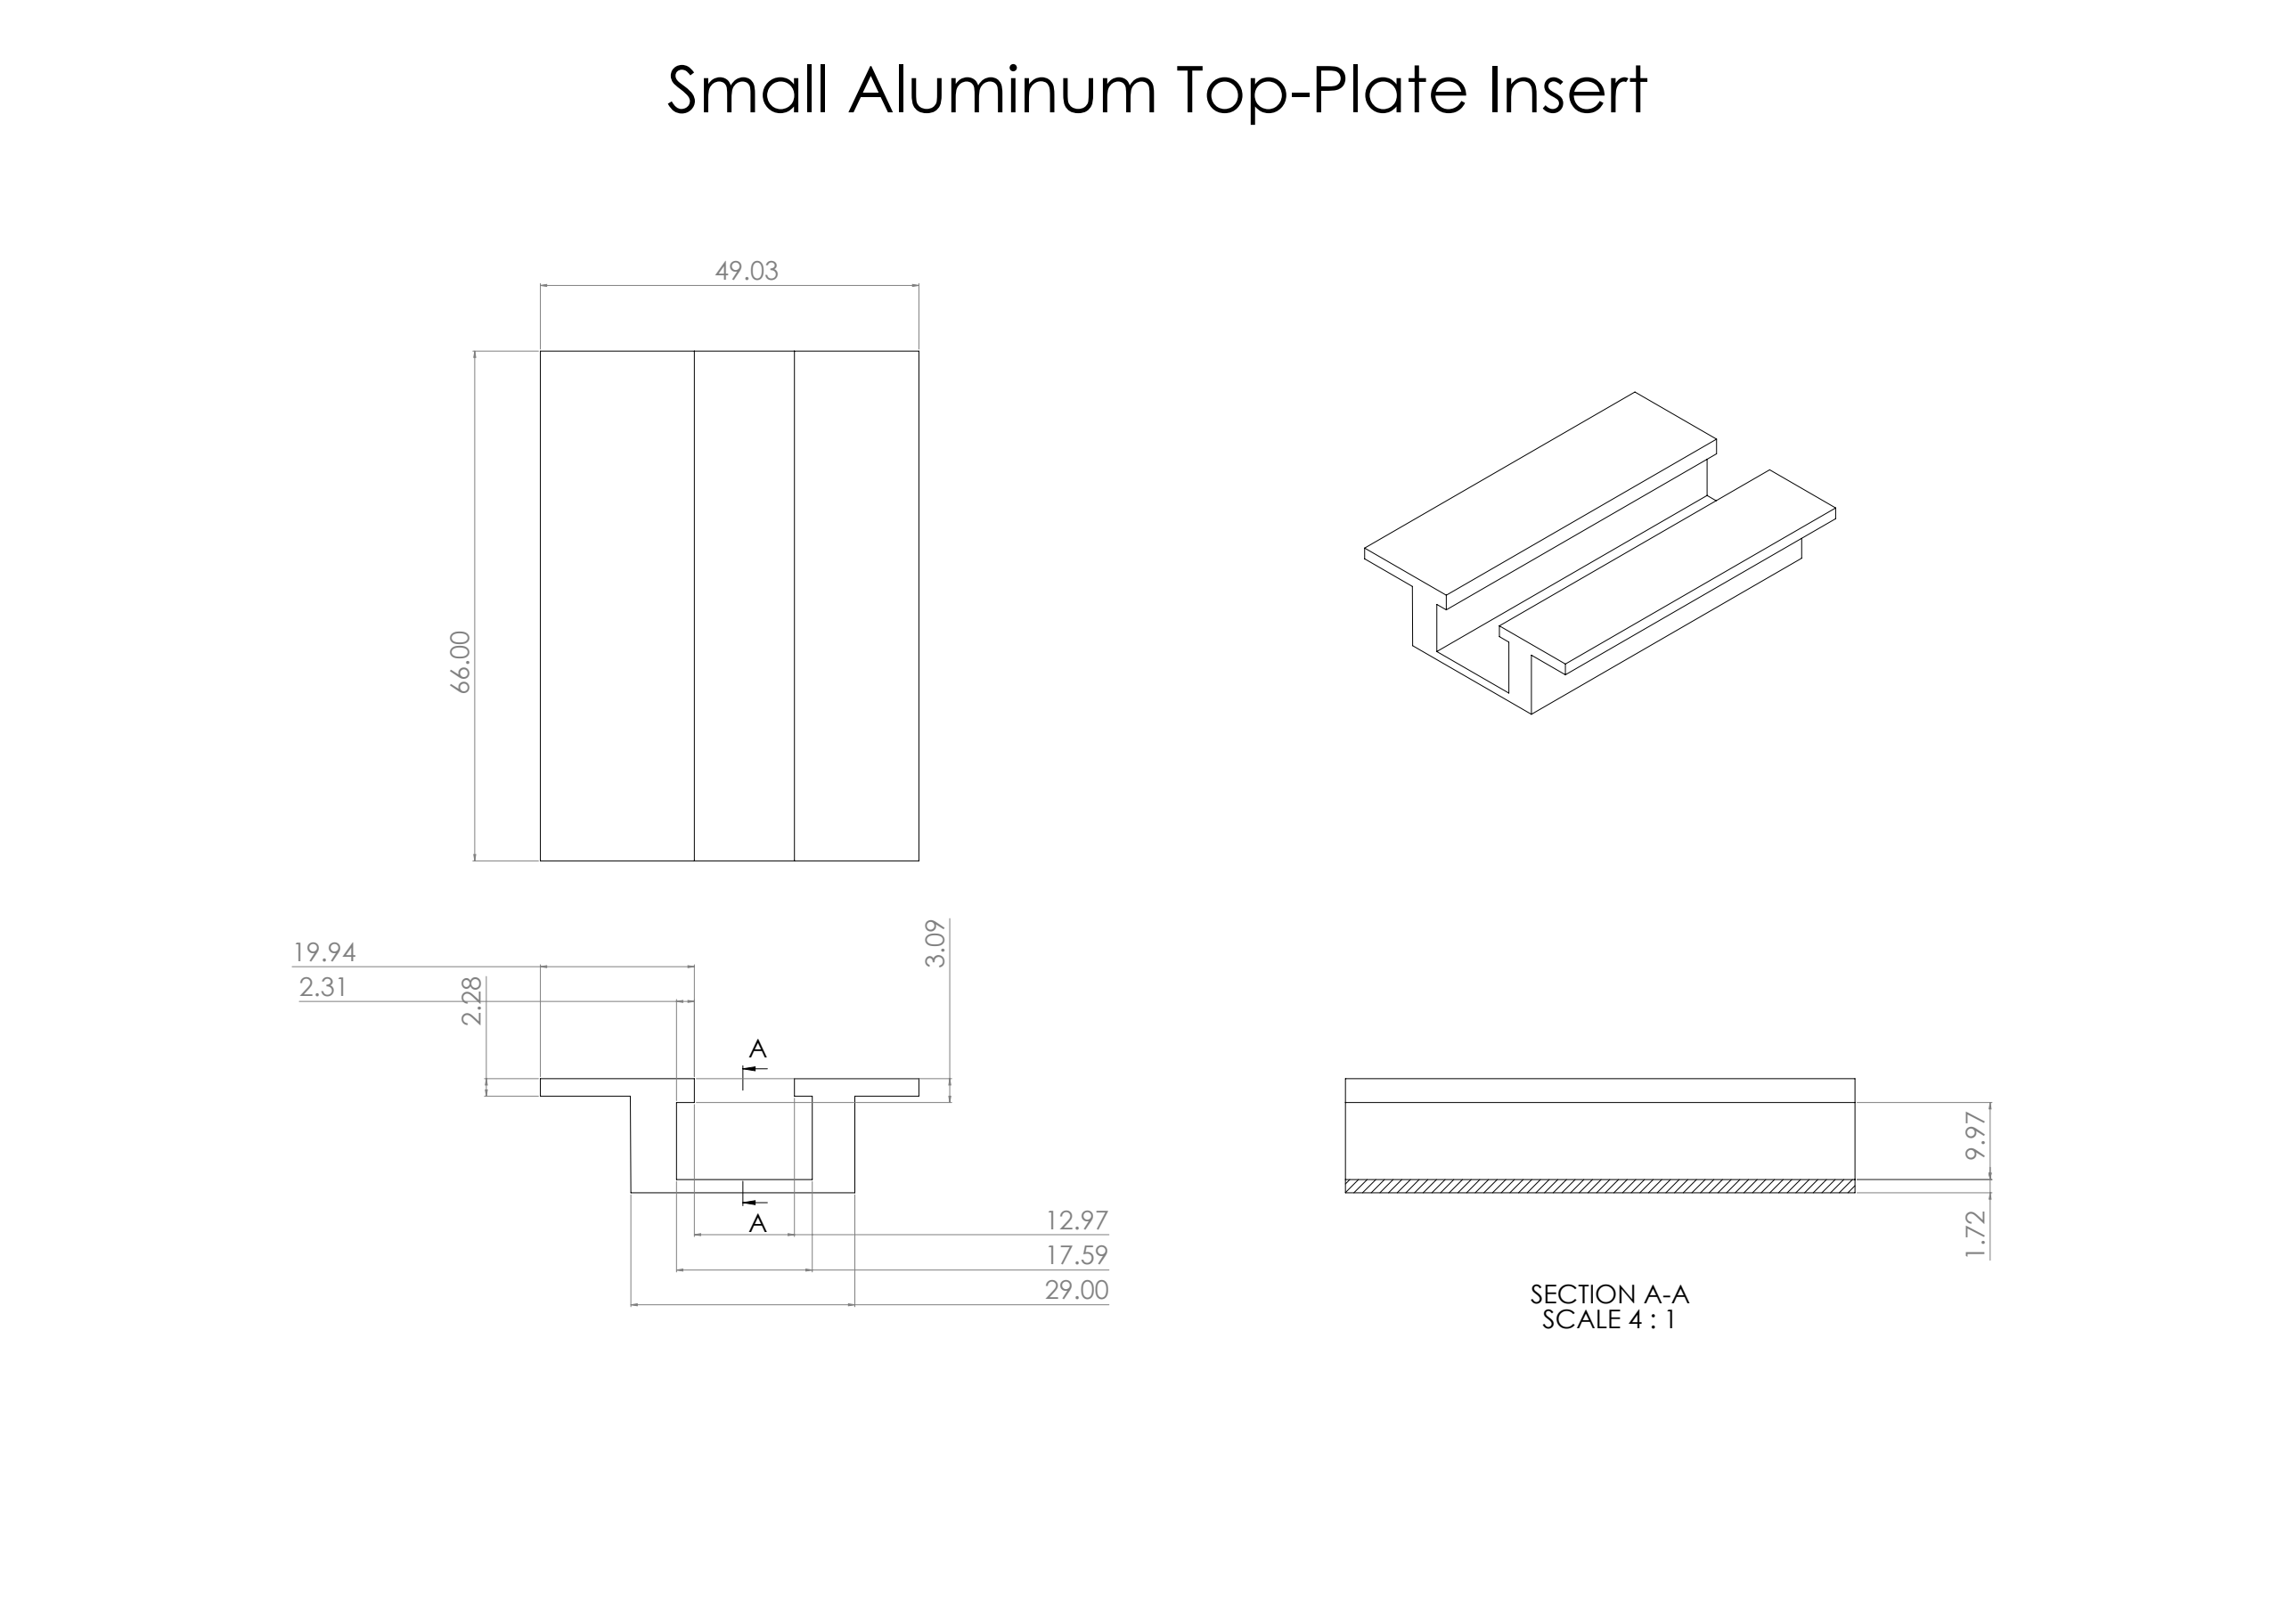
ISO-10303-21;
HEADER;
FILE_DESCRIPTION (('STEP AP214'),
    '1' );
FILE_NAME ('Small Aluminum Top-Plate Insert.step',
    '2026-10-24T21:31:31',
    ( '' ),
    ( '' ),
    'SwSTEP 2.0',
    'SolidWorks 2025',
    '' );
FILE_SCHEMA (( 'AUTOMOTIVE_DESIGN' ));
ENDSEC;

DATA;
#11=EDGE_LOOP ( 'NONE', ( #10298, #886, #9841, #4831, #11174, #11784, #1803, #163, #11627, #11601, #5374, #7472, #708, #12281, #12120, #14505 ) ) ;
#69=LINE ( 'NONE', #10606, #11985 ) ;
#101=ORIENTED_EDGE ( 'NONE', *, *, #8706, .F. ) ;
#123=ADVANCED_FACE ( 'NONE', ( #3273 ), #5820, .F. ) ;
#148=LINE ( 'NONE', #14233, #12794 ) ;
#163=ORIENTED_EDGE ( 'NONE', *, *, #14073, .T. ) ;
#171=VECTOR ( 'NONE', #13826, 1000.000000000000000 ) ;
#187=CARTESIAN_POINT ( 'NONE',  ( 67.21328690825531282, 25.52935533987996664, 84.20452624982236500 ) ) ;
#212=PLANE ( 'NONE',  #10140 ) ;
#275=AXIS2_PLACEMENT_3D ( 'NONE', #4169, #10894, #7496 ) ;
#346=LINE ( 'NONE', #12902, #10507 ) ;
#348=CARTESIAN_POINT ( 'NONE',  ( 96.29968967959054282, 25.52935533987996664, 33.00000000000012790 ) ) ;
#409=EDGE_CURVE ( 'NONE', #4378, #2618, #11532, .T. ) ;
#440=CARTESIAN_POINT ( 'NONE',  ( 96.29968967959054282, 23.25070940071369208, 33.00000000000012790 ) ) ;
#479=EDGE_LOOP ( 'NONE', ( #6850, #11834, #11522, #3223 ) ) ;
#480=CARTESIAN_POINT ( 'NONE',  ( 88.00000000000001421, 10.75070940071369208, -33.00000000000012790 ) ) ;
#488=CARTESIAN_POINT ( 'NONE',  ( 47.27423575335444639, 23.25070940071368852, 84.20452624982236500 ) ) ;
#497=FACE_OUTER_BOUND ( 'NONE', #6933, .T. ) ;
#563=LINE ( 'NONE', #7876, #12055 ) ;
#591=DIRECTION ( 'NONE',  ( -1.000000000000000000, 0.000000000000000000, 0.000000000000000000 ) ) ;
#619=VERTEX_POINT ( 'NONE', #7390 ) ;
#630=AXIS2_PLACEMENT_3D ( 'NONE', #11136, #591, #8901 ) ;
#654=ADVANCED_FACE ( 'NONE', ( #5008 ), #9713, .F. ) ;
#676=VECTOR ( 'NONE', #14030, 1000.000000000000000 ) ;
#698=DIRECTION ( 'NONE',  ( 0.000000000000000000, -1.000000000000000000, 0.000000000000000000 ) ) ;
#708=ORIENTED_EDGE ( 'NONE', *, *, #10704, .T. ) ;
#734=CARTESIAN_POINT ( 'NONE',  ( 67.21328690825531282, 25.52935533987996664, -33.00000000000012790 ) ) ;
#750=VERTEX_POINT ( 'NONE', #6949 ) ;
#765=DIRECTION ( 'NONE',  ( 0.000000000000000000, -1.000000000000000000, 0.000000000000000000 ) ) ;
#770=VECTOR ( 'NONE', #9472, 1000.000000000000000 ) ;
#788=VERTEX_POINT ( 'NONE', #4558 ) ;
#803=VECTOR ( 'NONE', #6520, 1000.000000000000000 ) ;
#823=CARTESIAN_POINT ( 'NONE',  ( 80.18290120114222930, 25.52935533987996664, 84.20452624982236500 ) ) ;
#848=ORIENTED_EDGE ( 'NONE', *, *, #10704, .F. ) ;
#878=CARTESIAN_POINT ( 'NONE',  ( 82.49066175147797253, 12.46743062497963450, -33.00000000000012790 ) ) ;
#886=ORIENTED_EDGE ( 'NONE', *, *, #4268, .T. ) ;
#895=VECTOR ( 'NONE', #2862, 1000.000000000000000 ) ;
#923=VECTOR ( 'NONE', #12640, 1000.000000000000000 ) ;
#929=SHAPE_REPRESENTATION_RELATIONSHIP ( 'NONE' , 'NONE' ,  #2449, #8343 ) ;
#949=EDGE_CURVE ( 'NONE', #3754, #3249, #2996, .T. ) ;
#962=AXIS2_PLACEMENT_3D ( 'NONE', #12322, #765, #7710 ) ;
#969=EDGE_CURVE ( 'NONE', #12642, #2618, #1832, .T. ) ;
#1004=STYLED_ITEM('',(#15279),#4097);
#1041=VECTOR ( 'NONE', #698, 1000.000000000000000 ) ;
#1096=VERTEX_POINT ( 'NONE', #9302 ) ;
#1101=LINE ( 'NONE', #5813, #11583 ) ;
#1148=CARTESIAN_POINT ( 'NONE',  ( 88.00000000000000000, 23.25070940071369208, -33.00000000000012790 ) ) ;
#1158=DIRECTION ( 'NONE',  ( -1.110223024625156540E-15, 1.000000000000000000, 0.000000000000000000 ) ) ;
#1177=EDGE_CURVE ( 'NONE', #9470, #12642, #1669, .T. ) ;
#1199=PRODUCT_DEFINITION ( 'UNKNOWN', '', #11005, #4748 ) ;
#1215=ORIENTED_EDGE ( 'NONE', *, *, #949, .F. ) ;
#1218=ORIENTED_EDGE ( 'NONE', *, *, #5311, .F. ) ;
#1279=PLANE ( 'NONE',  #11718 ) ;
#1339=LINE ( 'NONE', #187, #12832 ) ;
#1347=DIRECTION ( 'NONE',  ( -0.000000000000000000, -0.000000000000000000, -1.000000000000000000 ) ) ;
#1354=ORIENTED_EDGE ( 'NONE', *, *, #14964, .T. ) ;
#1356=ORIENTED_EDGE ( 'NONE', *, *, #9741, .T. ) ;
#1369=CARTESIAN_POINT ( 'NONE',  ( 59.06137132172460014, 0.3483485318593032565, -33.00000000000012790 ) ) ;
#1378=ORIENTED_EDGE ( 'NONE', *, *, #14002, .T. ) ;
#1387=ADVANCED_FACE ( 'NONE', ( #12279 ), #6653, .F. ) ;
#1433=EDGE_LOOP ( 'NONE', ( #6266, #13083, #3751, #10819 ) ) ;
#1441=VERTEX_POINT ( 'NONE', #10128 ) ;
#1474=VERTEX_POINT ( 'NONE', #878 ) ;
#1497=LINE ( 'NONE', #348, #6923 ) ;
#1509=ORIENTED_EDGE ( 'NONE', *, *, #11188, .T. ) ;
#1516=ORIENTED_EDGE ( 'NONE', *, *, #409, .F. ) ;
#1536=LINE ( 'NONE', #2764, #13361 ) ;
#1538=VECTOR ( 'NONE', #4607, 1000.000000000000000 ) ;
#1539=VECTOR ( 'NONE', #8765, 1000.000000000000000 ) ;
#1541=ORIENTED_EDGE ( 'NONE', *, *, #13654, .F. ) ;
#1562=CARTESIAN_POINT ( 'NONE',  ( 67.21328690825531282, 22.43695620243006772, -33.00000000000012790 ) ) ;
#1586=CARTESIAN_POINT ( 'NONE',  ( 58.92629142760363692, 23.25070940071368852, 84.20452624982236500 ) ) ;
#1598=ORIENTED_EDGE ( 'NONE', *, *, #5035, .T. ) ;
#1660=PLANE ( 'NONE',  #10735 ) ;
#1669=LINE ( 'NONE', #12057, #6239 ) ;
#1709=DIRECTION ( 'NONE',  ( -1.000000000000000000, -1.156482317317871725E-16, 0.000000000000000000 ) ) ;
#1739=EDGE_CURVE ( 'NONE', #6140, #7395, #10489, .T. ) ;
#1803=ORIENTED_EDGE ( 'NONE', *, *, #5053, .T. ) ;
#1832=LINE ( 'NONE', #823, #803 ) ;
#1899=ORIENTED_EDGE ( 'NONE', *, *, #14964, .F. ) ;
#1930=ORIENTED_EDGE ( 'NONE', *, *, #9241, .F. ) ;
#1931=( NAMED_UNIT ( * ) PLANE_ANGLE_UNIT ( ) SI_UNIT ( $, .RADIAN. ) );
#1947=DIRECTION ( 'NONE',  ( -0.000000000000000000, -0.000000000000000000, -1.000000000000000000 ) ) ;
#1949=VECTOR ( 'NONE', #5608, 1000.000000000000000 ) ;
#1954=DIRECTION ( 'NONE',  ( 0.000000000000000000, -1.000000000000000000, 0.000000000000000000 ) ) ;
#1969=EDGE_CURVE ( 'NONE', #11430, #3386, #11495, .T. ) ;
#1982=ORIENTED_EDGE ( 'NONE', *, *, #1177, .F. ) ;
#1986=VECTOR ( 'NONE', #11667, 1000.000000000000000 ) ;
#2001=APPLICATION_CONTEXT ( 'automotive_design' ) ;
#2023=EDGE_LOOP ( 'NONE', ( #2080, #1378, #2516, #4174 ) ) ;
#2048=ORIENTED_EDGE ( 'NONE', *, *, #14002, .F. ) ;
#2065=ORIENTED_EDGE ( 'NONE', *, *, #2181, .T. ) ;
#2071=CARTESIAN_POINT ( 'NONE',  ( 96.29968967959054282, 25.52935533987996664, -33.00000000000012790 ) ) ;
#2080=ORIENTED_EDGE ( 'NONE', *, *, #9815, .F. ) ;
#2129=( GEOMETRIC_REPRESENTATION_CONTEXT ( 3 ) GLOBAL_UNCERTAINTY_ASSIGNED_CONTEXT ( ( #13980 ) ) GLOBAL_UNIT_ASSIGNED_CONTEXT ( ( #12561, #1931, #12718 ) ) REPRESENTATION_CONTEXT ( 'NONE', 'WORKASPACE' ) );
#2181=EDGE_CURVE ( 'NONE', #9470, #5069, #5821, .T. ) ;
#2237=ORIENTED_EDGE ( 'NONE', *, *, #6729, .T. ) ;
#2276=VECTOR ( 'NONE', #5661, 1000.000000000000000 ) ;
#2347=DIRECTION ( 'NONE',  ( 0.000000000000000000, 0.000000000000000000, 1.000000000000000000 ) ) ;
#2363=CARTESIAN_POINT ( 'NONE',  ( 57.92627403409715470, 23.25070940071368852, -33.00000000000012790 ) ) ;
#2366=ORIENTED_EDGE ( 'NONE', *, *, #14128, .F. ) ;
#2443=APPLICATION_CONTEXT ( 'automotive_design' ) ;
#2449=SHAPE_REPRESENTATION ( 'Small Aluminum Top-Plate Insert', ( #6315 ), #2129 ) ;
#2461=CARTESIAN_POINT ( 'NONE',  ( 64.90552635791956959, 12.46743062497963450, -33.00000000000012790 ) ) ;
#2516=ORIENTED_EDGE ( 'NONE', *, *, #9344, .F. ) ;
#2553=AXIS2_PLACEMENT_3D ( 'NONE', #10050, #14815, #4114 ) ;
#2618=VERTEX_POINT ( 'NONE', #6600 ) ;
#2656=EDGE_CURVE ( 'NONE', #9890, #6001, #8753, .T. ) ;
#2722=DIRECTION ( 'NONE',  ( 0.000000000000000000, -1.000000000000000000, 0.000000000000000000 ) ) ;
#2764=CARTESIAN_POINT ( 'NONE',  ( 67.21328690825531282, 25.52935533987996664, 33.00000000000012790 ) ) ;
#2799=LINE ( 'NONE', #7492, #3177 ) ;
#2814=CARTESIAN_POINT ( 'NONE',  ( 82.49066175147797253, 23.25070940071369208, -33.00000000000012790 ) ) ;
#2862=DIRECTION ( 'NONE',  ( -0.000000000000000000, -0.000000000000000000, -1.000000000000000000 ) ) ;
#2867=PLANE ( 'NONE',  #10844 ) ;
#2887=VERTEX_POINT ( 'NONE', #8441 ) ;
#2913=DIRECTION ( 'NONE',  ( -1.000000000000000000, 0.000000000000000000, 0.000000000000000000 ) ) ;
#2942=ADVANCED_FACE ( 'NONE', ( #8574 ), #14429, .F. ) ;
#2951=ADVANCED_FACE ( 'NONE', ( #13565 ), #2867, .F. ) ;
#2964=ORIENTED_EDGE ( 'NONE', *, *, #7226, .F. ) ;
#2966=DIRECTION ( 'NONE',  ( -0.000000000000000000, 0.000000000000000000, 1.000000000000000000 ) ) ;
#2981=ORIENTED_EDGE ( 'NONE', *, *, #4998, .F. ) ;
#2996=LINE ( 'NONE', #5610, #10659 ) ;
#3008=ADVANCED_FACE ( 'NONE', ( #4019 ), #7425, .F. ) ;
#3038=DIRECTION ( 'NONE',  ( 0.000000000000000000, 0.000000000000000000, 1.000000000000000000 ) ) ;
#3087=CARTESIAN_POINT ( 'NONE',  ( 88.00000000000001421, 10.75070940071369208, 33.00000000000012790 ) ) ;
#3092=CARTESIAN_POINT ( 'NONE',  ( 47.27423575335444639, 23.25070940071368852, 33.00000000000012790 ) ) ;
#3172=VERTEX_POINT ( 'NONE', #10649 ) ;
#3177=VECTOR ( 'NONE', #12177, 1000.000000000000000 ) ;
#3223=ORIENTED_EDGE ( 'NONE', *, *, #6729, .F. ) ;
#3249=VERTEX_POINT ( 'NONE', #8268 ) ;
#3270=DIRECTION ( 'NONE',  ( -1.000000000000000000, 0.000000000000000000, 0.000000000000000000 ) ) ;
#3273=FACE_OUTER_BOUND ( 'NONE', #9368, .T. ) ;
#3290=DIRECTION ( 'NONE',  ( -0.005897974685767391929, 0.9999826067960413400, 0.000000000000000000 ) ) ;
#3293=LINE ( 'NONE', #13605, #1949 ) ;
#3386=VERTEX_POINT ( 'NONE', #1562 ) ;
#3462=PLANE ( 'NONE',  #6224 ) ;
#3465=LINE ( 'NONE', #1148, #770 ) ;
#3528=ADVANCED_FACE ( 'NONE', ( #12252 ), #6539, .F. ) ;
#3591=DIRECTION ( 'NONE',  ( 0.000000000000000000, 1.000000000000000000, -0.000000000000000000 ) ) ;
#3624=ORIENTED_EDGE ( 'NONE', *, *, #2656, .T. ) ;
#3677=EDGE_CURVE ( 'NONE', #3754, #788, #9224, .T. ) ;
#3690=EDGE_CURVE ( 'NONE', #6772, #1096, #3293, .T. ) ;
#3723=LINE ( 'NONE', #9670, #895 ) ;
#3751=ORIENTED_EDGE ( 'NONE', *, *, #5035, .F. ) ;
#3754=VERTEX_POINT ( 'NONE', #4438 ) ;
#3811=DIRECTION ( 'NONE',  ( 1.000000000000000000, 0.000000000000000000, 0.000000000000000000 ) ) ;
#3843=ORIENTED_EDGE ( 'NONE', *, *, #8706, .T. ) ;
#3898=CARTESIAN_POINT ( 'NONE',  ( 59.00001739350650354, 10.75070940071368852, 33.00000000000012790 ) ) ;
#3907=DIRECTION ( 'NONE',  ( -0.000000000000000000, -0.000000000000000000, -1.000000000000000000 ) ) ;
#3928=LINE ( 'NONE', #12242, #1539 ) ;
#3991=AXIS2_PLACEMENT_3D ( 'NONE', #6880, #3270, #4258 ) ;
#4019=FACE_OUTER_BOUND ( 'NONE', #7636, .T. ) ;
#4021=EDGE_CURVE ( 'NONE', #6859, #5990, #7026, .T. ) ;
#4024=ORIENTED_EDGE ( 'NONE', *, *, #11631, .T. ) ;
#4039=CARTESIAN_POINT ( 'NONE',  ( 96.29968967959054282, 25.52935533987996664, 84.20452624982236500 ) ) ;
#4059=DIRECTION ( 'NONE',  ( 0.000000000000000000, 1.000000000000000000, -0.000000000000000000 ) ) ;
#4079=EDGE_LOOP ( 'NONE', ( #9449, #4802, #6054, #101 ) ) ;
#4082=CARTESIAN_POINT ( 'NONE',  ( 0.000000000000000000, 0.000000000000000000, 0.000000000000000000 ) ) ;
#4097=MANIFOLD_SOLID_BREP ( 'Move Face2', #11190 ) ;
#4114=DIRECTION ( 'NONE',  ( 0.000000000000000000, -0.000000000000000000, -1.000000000000000000 ) ) ;
#4169=CARTESIAN_POINT ( 'NONE',  ( 88.00000000000000000, 23.25070940071369208, 84.20452624982236500 ) ) ;
#4174=ORIENTED_EDGE ( 'NONE', *, *, #10349, .F. ) ;
#4222=CARTESIAN_POINT ( 'NONE',  ( 82.49066175147797253, 23.25070940071369208, 33.00000000000012790 ) ) ;
#4244=PRODUCT_DEFINITION_SHAPE ( 'NONE', 'NONE',  #1199 ) ;
#4258=DIRECTION ( 'NONE',  ( 0.000000000000000000, 0.000000000000000000, 1.000000000000000000 ) ) ;
#4268=EDGE_CURVE ( 'NONE', #5864, #9470, #1497, .T. ) ;
#4360=VECTOR ( 'NONE', #1954, 1000.000000000000000 ) ;
#4378=VERTEX_POINT ( 'NONE', #11617 ) ;
#4438=CARTESIAN_POINT ( 'NONE',  ( 82.49066175147797253, 23.25070940071369208, 33.00000000000014211 ) ) ;
#4452=DIRECTION ( 'NONE',  ( 1.000000000000000000, -0.000000000000000000, 0.000000000000000000 ) ) ;
#4519=EDGE_CURVE ( 'NONE', #6001, #619, #3465, .T. ) ;
#4558=CARTESIAN_POINT ( 'NONE',  ( 82.49066175147797253, 23.25070940071369208, -33.00000000000012790 ) ) ;
#4564=CARTESIAN_POINT ( 'NONE',  ( 59.00001739350650354, 10.75070940071368852, 84.20452624982236500 ) ) ;
#4588=ORIENTED_EDGE ( 'NONE', *, *, #14888, .F. ) ;
#4607=DIRECTION ( 'NONE',  ( -0.000000000000000000, -0.000000000000000000, -1.000000000000000000 ) ) ;
#4614=DIRECTION ( 'NONE',  ( 1.000000000000000000, -0.000000000000000000, 0.000000000000000000 ) ) ;
#4627=VERTEX_POINT ( 'NONE', #9183 ) ;
#4629=EDGE_CURVE ( 'NONE', #14228, #1441, #10415, .T. ) ;
#4743=VECTOR ( 'NONE', #14648, 1000.000000000000000 ) ;
#4748=PRODUCT_DEFINITION_CONTEXT ( 'detailed design', #2001, 'design' ) ;
#4771=ORIENTED_EDGE ( 'NONE', *, *, #7741, .F. ) ;
#4802=ORIENTED_EDGE ( 'NONE', *, *, #12107, .T. ) ;
#4818=ORIENTED_EDGE ( 'NONE', *, *, #14852, .F. ) ;
#4831=ORIENTED_EDGE ( 'NONE', *, *, #4998, .T. ) ;
#4842=CARTESIAN_POINT ( 'NONE',  ( -16.99999999999998579, -2.249290599286303927, 33.00000000000012790 ) ) ;
#4998=EDGE_CURVE ( 'NONE', #12642, #2887, #3928, .T. ) ;
#5008=FACE_OUTER_BOUND ( 'NONE', #14284, .T. ) ;
#5034=CARTESIAN_POINT ( 'NONE',  ( 80.18290120114222930, 23.25070940071369208, 84.20452624982236500 ) ) ;
#5035=EDGE_CURVE ( 'NONE', #5069, #9890, #6184, .T. ) ;
#5053=EDGE_CURVE ( 'NONE', #3249, #12316, #8697, .T. ) ;
#5069=VERTEX_POINT ( 'NONE', #2071 ) ;
#5087=EDGE_CURVE ( 'NONE', #2887, #3754, #13770, .T. ) ;
#5088=EDGE_LOOP ( 'NONE', ( #2964, #14634, #9945, #10176 ) ) ;
#5127=CARTESIAN_POINT ( 'NONE',  ( 88.00000000000000000, 23.25070940071369208, 33.00000000000014211 ) ) ;
#5133=DIRECTION ( 'NONE',  ( 1.000000000000000000, -0.000000000000000000, 0.000000000000000000 ) ) ;
#5171=ADVANCED_FACE ( 'NONE', ( #11612 ), #3462, .T. ) ;
#5196=CARTESIAN_POINT ( 'NONE',  ( 0.000000000000000000, 0.000000000000000000, -33.00000000000012790 ) ) ;
#5206=ORIENTED_EDGE ( 'NONE', *, *, #409, .T. ) ;
#5209=PLANE ( 'NONE',  #14912 ) ;
#5218=CARTESIAN_POINT ( 'NONE',  ( 64.90552635791956959, 22.43695620243006772, -33.00000000000012790 ) ) ;
#5231=PLANE ( 'NONE',  #13467 ) ;
#5276=DIRECTION ( 'NONE',  ( 1.000000000000000000, 0.000000000000000000, 0.000000000000000000 ) ) ;
#5311=EDGE_CURVE ( 'NONE', #1096, #14996, #1536, .T. ) ;
#5326=EDGE_CURVE ( 'NONE', #750, #4627, #6374, .T. ) ;
#5352=CARTESIAN_POINT ( 'NONE',  ( 67.21328690825531282, 25.52935533987996664, -33.00000000000012790 ) ) ;
#5374=ORIENTED_EDGE ( 'NONE', *, *, #9815, .T. ) ;
#5447=CARTESIAN_POINT ( 'NONE',  ( 58.99998260679605266, 10.75660737539945622, 84.20452624982236500 ) ) ;
#5466=VECTOR ( 'NONE', #6324, 1000.000000000000000 ) ;
#5510=CARTESIAN_POINT ( 'NONE',  ( 80.18290120114222930, 25.52935533987996664, -33.00000000000012790 ) ) ;
#5562=ORIENTED_EDGE ( 'NONE', *, *, #14852, .T. ) ;
#5605=DIRECTION ( 'NONE',  ( 0.9999826067960413400, 0.005897974685767391929, -0.000000000000000000 ) ) ;
#5608=DIRECTION ( 'NONE',  ( 1.000000000000000000, -0.000000000000000000, 0.000000000000000000 ) ) ;
#5610=CARTESIAN_POINT ( 'NONE',  ( 82.49066175147797253, 12.46743062497963450, 33.00000000000012790 ) ) ;
#5646=DIRECTION ( 'NONE',  ( 0.005897974685767391929, -0.9999826067960413400, 0.000000000000000000 ) ) ;
#5661=DIRECTION ( 'NONE',  ( 1.000000000000000000, -0.000000000000000000, 0.000000000000000000 ) ) ;
#5671=VECTOR ( 'NONE', #14857, 1000.000000000000000 ) ;
#5715=CARTESIAN_POINT ( 'NONE',  ( 88.00000000000000000, 23.25070940071369208, 33.00000000000012790 ) ) ;
#5747=PLANE ( 'NONE',  #3991 ) ;
#5767=CARTESIAN_POINT ( 'NONE',  ( 47.27423575335444639, 25.52935533987996664, 33.00000000000012790 ) ) ;
#5813=CARTESIAN_POINT ( 'NONE',  ( 64.90552635791956959, 22.43695620243006772, 33.00000000000012790 ) ) ;
#5820=PLANE ( 'NONE',  #6330 ) ;
#5821=LINE ( 'NONE', #15203, #13975 ) ;
#5831=VECTOR ( 'NONE', #3907, 1000.000000000000000 ) ;
#5864=VERTEX_POINT ( 'NONE', #13259 ) ;
#5913=ORIENTED_EDGE ( 'NONE', *, *, #3677, .T. ) ;
#5990=VERTEX_POINT ( 'NONE', #6476 ) ;
#6001=VERTEX_POINT ( 'NONE', #6395 ) ;
#6043=PLANE ( 'NONE',  #13108 ) ;
#6054=ORIENTED_EDGE ( 'NONE', *, *, #8949, .F. ) ;
#6137=EDGE_LOOP ( 'NONE', ( #6525, #11863, #13007, #14651 ) ) ;
#6140=VERTEX_POINT ( 'NONE', #11696 ) ;
#6161=LINE ( 'NONE', #6240, #5831 ) ;
#6184=LINE ( 'NONE', #10870, #5466 ) ;
#6186=VECTOR ( 'NONE', #2913, 1000.000000000000000 ) ;
#6219=LINE ( 'NONE', #1586, #4743 ) ;
#6224=AXIS2_PLACEMENT_3D ( 'NONE', #4842, #14160, #8159 ) ;
#6239=VECTOR ( 'NONE', #8665, 1000.000000000000000 ) ;
#6240=CARTESIAN_POINT ( 'NONE',  ( 88.00000000000001421, 10.75070940071369208, 84.20452624982236500 ) ) ;
#6266=ORIENTED_EDGE ( 'NONE', *, *, #4268, .F. ) ;
#6315=AXIS2_PLACEMENT_3D ( 'NONE', #4082, #8567, #11096 ) ;
#6324=DIRECTION ( 'NONE',  ( 0.000000000000000000, -1.000000000000000000, 0.000000000000000000 ) ) ;
#6330=AXIS2_PLACEMENT_3D ( 'NONE', #10282, #9356, #2347 ) ;
#6374=LINE ( 'NONE', #5218, #9407 ) ;
#6383=FACE_OUTER_BOUND ( 'NONE', #4079, .T. ) ;
#6395=CARTESIAN_POINT ( 'NONE',  ( 88.00000000000000000, 23.25070940071369208, -33.00000000000012790 ) ) ;
#6411=DIRECTION ( 'NONE',  ( 1.000000000000000000, 0.000000000000000000, 0.000000000000000000 ) ) ;
#6476=CARTESIAN_POINT ( 'NONE',  ( 59.00001739350650354, 10.75070940071368852, -33.00000000000012790 ) ) ;
#6520=DIRECTION ( 'NONE',  ( -0.000000000000000000, -0.000000000000000000, -1.000000000000000000 ) ) ;
#6525=ORIENTED_EDGE ( 'NONE', *, *, #14073, .F. ) ;
#6539=PLANE ( 'NONE',  #962 ) ;
#6600=CARTESIAN_POINT ( 'NONE',  ( 80.18290120114222930, 25.52935533987996664, -33.00000000000014211 ) ) ;
#6607=CARTESIAN_POINT ( 'NONE',  ( 64.90552635791956959, 12.46743062497963450, 84.20452624982236500 ) ) ;
#6653=PLANE ( 'NONE',  #2553 ) ;
#6729=EDGE_CURVE ( 'NONE', #1441, #6140, #69, .T. ) ;
#6746=ORIENTED_EDGE ( 'NONE', *, *, #4021, .T. ) ;
#6772=VERTEX_POINT ( 'NONE', #14379 ) ;
#6774=LINE ( 'NONE', #5715, #14186 ) ;
#6787=CARTESIAN_POINT ( 'NONE',  ( 58.99998260679605266, 10.75660737539945622, 33.00000000000012790 ) ) ;
#6850=ORIENTED_EDGE ( 'NONE', *, *, #4629, .F. ) ;
#6859=VERTEX_POINT ( 'NONE', #3898 ) ;
#6880=CARTESIAN_POINT ( 'NONE',  ( 67.21328690825531282, 25.52935533987996664, 84.20452624982236500 ) ) ;
#6923=VECTOR ( 'NONE', #10962, 1000.000000000000000 ) ;
#6933=EDGE_LOOP ( 'NONE', ( #1218, #3843, #14227, #2048 ) ) ;
#6946=EDGE_CURVE ( 'NONE', #14830, #5864, #10982, .T. ) ;
#6949=CARTESIAN_POINT ( 'NONE',  ( 64.90552635791956959, 22.43695620243006772, -33.00000000000012790 ) ) ;
#6950=VECTOR ( 'NONE', #4452, 1000.000000000000000 ) ;
#6995=VERTEX_POINT ( 'NONE', #13662 ) ;
#7026=LINE ( 'NONE', #4564, #14299 ) ;
#7036=FACE_OUTER_BOUND ( 'NONE', #7219, .T. ) ;
#7054=DIRECTION ( 'NONE',  ( 0.000000000000000000, 0.000000000000000000, -1.000000000000000000 ) ) ;
#7073=ORIENTED_EDGE ( 'NONE', *, *, #11338, .F. ) ;
#7077=ORIENTED_EDGE ( 'NONE', *, *, #8626, .F. ) ;
#7131=CARTESIAN_POINT ( 'NONE',  ( 82.49066175147797253, 12.46743062497963450, -33.00000000000012790 ) ) ;
#7219=EDGE_LOOP ( 'NONE', ( #7077, #6746, #2366, #7073 ) ) ;
#7226=EDGE_CURVE ( 'NONE', #11898, #14830, #6774, .T. ) ;
#7390=CARTESIAN_POINT ( 'NONE',  ( 88.00000000000001421, 10.75070940071369208, -33.00000000000012790 ) ) ;
#7395=VERTEX_POINT ( 'NONE', #14839 ) ;
#7401=CARTESIAN_POINT ( 'NONE',  ( 64.90552635791956959, 12.46743062497963450, 33.00000000000012790 ) ) ;
#7403=DIRECTION ( 'NONE',  ( -0.000000000000000000, -0.000000000000000000, -1.000000000000000000 ) ) ;
#7425=PLANE ( 'NONE',  #15010 ) ;
#7437=ORIENTED_EDGE ( 'NONE', *, *, #14754, .F. ) ;
#7453=LINE ( 'NONE', #1369, #10000 ) ;
#7471=ORIENTED_EDGE ( 'NONE', *, *, #14754, .T. ) ;
#7472=ORIENTED_EDGE ( 'NONE', *, *, #4629, .T. ) ;
#7487=ADVANCED_FACE ( 'NONE', ( #6383 ), #5231, .F. ) ;
#7492=CARTESIAN_POINT ( 'NONE',  ( 47.27423575335444639, 25.52935533987996664, -33.00000000000012790 ) ) ;
#7496=DIRECTION ( 'NONE',  ( 1.110223024625156540E-15, -1.000000000000000000, 0.000000000000000000 ) ) ;
#7505=EDGE_LOOP ( 'NONE', ( #1598, #3624, #9389, #13880, #7769, #1356, #14217, #9768, #10761, #14873, #12093, #1509, #12343, #5562, #5206, #8580 ) ) ;
#7569=DIRECTION ( 'NONE',  ( -1.000000000000000000, 0.000000000000000000, 0.000000000000000000 ) ) ;
#7636=EDGE_LOOP ( 'NONE', ( #1982, #2065, #4588, #9428 ) ) ;
#7710=DIRECTION ( 'NONE',  ( 0.000000000000000000, -0.000000000000000000, -1.000000000000000000 ) ) ;
#7736=FACE_OUTER_BOUND ( 'NONE', #7505, .T. ) ;
#7741=EDGE_CURVE ( 'NONE', #5990, #3172, #7453, .T. ) ;
#7745=DIRECTION ( 'NONE',  ( 0.000000000000000000, 0.000000000000000000, 1.000000000000000000 ) ) ;
#7769=ORIENTED_EDGE ( 'NONE', *, *, #7741, .T. ) ;
#7835=PLANE ( 'NONE',  #11089 ) ;
#7868=ADVANCED_FACE ( 'NONE', ( #9979 ), #5209, .F. ) ;
#7876=CARTESIAN_POINT ( 'NONE',  ( 67.21328690825531282, 22.43695620243006772, -33.00000000000012790 ) ) ;
#7917=DIRECTION ( 'NONE',  ( -0.000000000000000000, -0.000000000000000000, -1.000000000000000000 ) ) ;
#7948=CARTESIAN_POINT ( 'NONE',  ( 57.92627403409715470, 23.25070940071368852, 33.00000000000012790 ) ) ;
#7951=CARTESIAN_POINT ( 'NONE',  ( 88.00000000000001421, 10.75070940071369208, 33.00000000000014211 ) ) ;
#8159=DIRECTION ( 'NONE',  ( 1.000000000000000000, 0.000000000000000000, -0.000000000000000000 ) ) ;
#8166=ADVANCED_FACE ( 'NONE', ( #8578 ), #12413, .F. ) ;
#8195=ORIENTED_EDGE ( 'NONE', *, *, #6946, .F. ) ;
#8268=CARTESIAN_POINT ( 'NONE',  ( 82.49066175147797253, 12.46743062497963450, 33.00000000000014211 ) ) ;
#8297=ORIENTED_EDGE ( 'NONE', *, *, #3677, .F. ) ;
#8343=ADVANCED_BREP_SHAPE_REPRESENTATION ( '', ( #4097, #6315 ), #2129 ) ;
#8441=CARTESIAN_POINT ( 'NONE',  ( 80.18290120114222930, 23.25070940071369208, 33.00000000000014211 ) ) ;
#8453=CARTESIAN_POINT ( 'NONE',  ( 82.49066175147797253, 12.46743062497963450, 84.20452624982236500 ) ) ;
#8454=DIRECTION ( 'NONE',  ( 0.000000000000000000, 0.000000000000000000, 1.000000000000000000 ) ) ;
#8567=DIRECTION ( 'NONE',  ( 0.000000000000000000, 0.000000000000000000, 1.000000000000000000 ) ) ;
#8574=FACE_OUTER_BOUND ( 'NONE', #5088, .T. ) ;
#8578=FACE_OUTER_BOUND ( 'NONE', #13560, .T. ) ;
#8580=ORIENTED_EDGE ( 'NONE', *, *, #14888, .T. ) ;
#8596=EDGE_LOOP ( 'NONE', ( #13225, #1354, #11012, #11705 ) ) ;
#8626=EDGE_CURVE ( 'NONE', #6859, #11898, #15018, .T. ) ;
#8632=VECTOR ( 'NONE', #1709, 1000.000000000000000 ) ;
#8654=CARTESIAN_POINT ( 'NONE',  ( 80.18290120114222930, 25.52935533987996664, 33.00000000000014211 ) ) ;
#8657=LINE ( 'NONE', #2814, #10643 ) ;
#8665=DIRECTION ( 'NONE',  ( -1.000000000000000000, 0.000000000000000000, 0.000000000000000000 ) ) ;
#8697=LINE ( 'NONE', #7401, #14802 ) ;
#8698=LINE ( 'NONE', #10950, #14632 ) ;
#8706=EDGE_CURVE ( 'NONE', #1096, #3386, #148, .T. ) ;
#8749=ORIENTED_EDGE ( 'NONE', *, *, #9741, .F. ) ;
#8750=VECTOR ( 'NONE', #4614, 1000.000000000000000 ) ;
#8753=LINE ( 'NONE', #13451, #6186 ) ;
#8757=DIRECTION ( 'NONE',  ( 0.000000000000000000, 0.000000000000000000, 1.000000000000000000 ) ) ;
#8765=DIRECTION ( 'NONE',  ( 0.000000000000000000, -1.000000000000000000, 0.000000000000000000 ) ) ;
#8860=CARTESIAN_POINT ( 'NONE',  ( 47.27423575335444639, 25.52935533987996664, 33.00000000000014211 ) ) ;
#8879=VECTOR ( 'NONE', #14270, 1000.000000000000000 ) ;
#8901=DIRECTION ( 'NONE',  ( 0.000000000000000000, 0.000000000000000000, 1.000000000000000000 ) ) ;
#8949=EDGE_CURVE ( 'NONE', #3386, #750, #563, .T. ) ;
#9022=AXIS2_PLACEMENT_3D ( 'NONE', #9781, #14395, #11999 ) ;
#9160=ORIENTED_EDGE ( 'NONE', *, *, #2656, .F. ) ;
#9183=CARTESIAN_POINT ( 'NONE',  ( 64.90552635791956959, 12.46743062497963450, -33.00000000000012790 ) ) ;
#9199=LINE ( 'NONE', #9349, #8879 ) ;
#9202=CARTESIAN_POINT ( 'NONE',  ( 67.21328690825531282, 25.52935533987996664, 33.00000000000014211 ) ) ;
#9224=LINE ( 'NONE', #13908, #9593 ) ;
#9241=EDGE_CURVE ( 'NONE', #6995, #6859, #15189, .T. ) ;
#9251=CARTESIAN_POINT ( 'NONE',  ( 96.29968967959054282, 25.52935533987996664, 33.00000000000014211 ) ) ;
#9277=EDGE_CURVE ( 'NONE', #2887, #4378, #13266, .T. ) ;
#9289=LINE ( 'NONE', #7131, #1986 ) ;
#9302=CARTESIAN_POINT ( 'NONE',  ( 67.21328690825531282, 22.43695620243006772, 33.00000000000014211 ) ) ;
#9344=EDGE_CURVE ( 'NONE', #7395, #11430, #2799, .T. ) ;
#9349=CARTESIAN_POINT ( 'NONE',  ( 96.29968967959054282, 23.25070940071369208, 84.20452624982236500 ) ) ;
#9356=DIRECTION ( 'NONE',  ( 0.000000000000000000, 1.000000000000000000, -0.000000000000000000 ) ) ;
#9368=EDGE_LOOP ( 'NONE', ( #848, #2237, #8749, #7437 ) ) ;
#9389=ORIENTED_EDGE ( 'NONE', *, *, #4519, .T. ) ;
#9407=VECTOR ( 'NONE', #10847, 1000.000000000000000 ) ;
#9428=ORIENTED_EDGE ( 'NONE', *, *, #969, .F. ) ;
#9449=ORIENTED_EDGE ( 'NONE', *, *, #3690, .F. ) ;
#9468=LINE ( 'NONE', #2461, #8750 ) ;
#9470=VERTEX_POINT ( 'NONE', #9251 ) ;
#9471=CARTESIAN_POINT ( 'NONE',  ( 64.90552635791956959, 12.46743062497963450, 33.00000000000014211 ) ) ;
#9472=DIRECTION ( 'NONE',  ( 1.110223024625156540E-15, -1.000000000000000000, 0.000000000000000000 ) ) ;
#9529=CARTESIAN_POINT ( 'NONE',  ( 96.29968967959054282, 23.25070940071369208, -33.00000000000012790 ) ) ;
#9593=VECTOR ( 'NONE', #7917, 1000.000000000000000 ) ;
#9594=VECTOR ( 'NONE', #9955, 1000.000000000000000 ) ;
#9657=ADVANCED_FACE ( 'NONE', ( #13437 ), #14826, .F. ) ;
#9670=CARTESIAN_POINT ( 'NONE',  ( 88.00000000000000000, 23.25070940071369208, 84.20452624982236500 ) ) ;
#9713=PLANE ( 'NONE',  #9022 ) ;
#9740=DIRECTION ( 'NONE',  ( -0.000000000000000000, -0.000000000000000000, -1.000000000000000000 ) ) ;
#9741=EDGE_CURVE ( 'NONE', #3172, #6140, #11672, .T. ) ;
#9744=CARTESIAN_POINT ( 'NONE',  ( 80.18290120114222930, 25.52935533987996664, 84.20452624982236500 ) ) ;
#9768=ORIENTED_EDGE ( 'NONE', *, *, #9344, .T. ) ;
#9781=CARTESIAN_POINT ( 'NONE',  ( 80.18290120114222930, 23.25070940071369208, 84.20452624982236500 ) ) ;
#9815=EDGE_CURVE ( 'NONE', #14996, #14228, #15138, .T. ) ;
#9841=ORIENTED_EDGE ( 'NONE', *, *, #1177, .T. ) ;
#9854=ADVANCED_FACE ( 'NONE', ( #13138 ), #1279, .F. ) ;
#9890=VERTEX_POINT ( 'NONE', #9529 ) ;
#9905=VECTOR ( 'NONE', #1947, 1000.000000000000000 ) ;
#9913=DIRECTION ( 'NONE',  ( -1.000000000000000000, 0.000000000000000000, 0.000000000000000000 ) ) ;
#9945=ORIENTED_EDGE ( 'NONE', *, *, #4519, .F. ) ;
#9955=DIRECTION ( 'NONE',  ( -0.000000000000000000, -0.000000000000000000, -1.000000000000000000 ) ) ;
#9979=FACE_OUTER_BOUND ( 'NONE', #1433, .T. ) ;
#10000=VECTOR ( 'NONE', #10837, 1000.000000000000000 ) ;
#10031=DIRECTION ( 'NONE',  ( 0.000000000000000000, 0.000000000000000000, -1.000000000000000000 ) ) ;
#10050=CARTESIAN_POINT ( 'NONE',  ( 64.90552635791956959, 12.46743062497963450, 84.20452624982236500 ) ) ;
#10054=ADVANCED_FACE ( 'NONE', ( #7736 ), #1660, .F. ) ;
#10128=CARTESIAN_POINT ( 'NONE',  ( 47.27423575335444639, 23.25070940071368852, 33.00000000000014211 ) ) ;
#10140=AXIS2_PLACEMENT_3D ( 'NONE', #8453, #3811, #7054 ) ;
#10176=ORIENTED_EDGE ( 'NONE', *, *, #11631, .F. ) ;
#10196=LINE ( 'NONE', #12420, #9905 ) ;
#10282=CARTESIAN_POINT ( 'NONE',  ( 57.92627403409715470, 23.25070940071368852, 84.20452624982236500 ) ) ;
#10298=ORIENTED_EDGE ( 'NONE', *, *, #6946, .T. ) ;
#10349=EDGE_CURVE ( 'NONE', #14228, #7395, #346, .T. ) ;
#10414=LINE ( 'NONE', #7948, #923 ) ;
#10415=LINE ( 'NONE', #3092, #1041 ) ;
#10489=LINE ( 'NONE', #14868, #676 ) ;
#10505=DIRECTION ( 'NONE',  ( -1.000000000000000000, -1.156482317317871725E-16, 0.000000000000000000 ) ) ;
#10507=VECTOR ( 'NONE', #9740, 1000.000000000000000 ) ;
#10582=DIRECTION ( 'NONE',  ( -1.156482317317871725E-16, 1.000000000000000000, 0.000000000000000000 ) ) ;
#10585=( NAMED_UNIT ( * ) SI_UNIT ( $, .STERADIAN. ) SOLID_ANGLE_UNIT ( ) );
#10606=CARTESIAN_POINT ( 'NONE',  ( 47.27423575335444639, 23.25070940071368852, 84.20452624982236500 ) ) ;
#10643=VECTOR ( 'NONE', #12192, 1000.000000000000000 ) ;
#10649=CARTESIAN_POINT ( 'NONE',  ( 58.92629142760364402, 23.25070940071368852, -33.00000000000012790 ) ) ;
#10659=VECTOR ( 'NONE', #14753, 1000.000000000000000 ) ;
#10677=FACE_OUTER_BOUND ( 'NONE', #14354, .T. ) ;
#10704=EDGE_CURVE ( 'NONE', #1441, #6995, #10414, .T. ) ;
#10735=AXIS2_PLACEMENT_3D ( 'NONE', #5196, #2966, #5276 ) ;
#10761=ORIENTED_EDGE ( 'NONE', *, *, #1969, .T. ) ;
#10765=VECTOR ( 'NONE', #5133, 1000.000000000000000 ) ;
#10819=ORIENTED_EDGE ( 'NONE', *, *, #2181, .F. ) ;
#10837=DIRECTION ( 'NONE',  ( -0.005897974685767391929, 0.9999826067960413400, 0.000000000000000000 ) ) ;
#10844=AXIS2_PLACEMENT_3D ( 'NONE', #488, #6411, #10031 ) ;
#10847=DIRECTION ( 'NONE',  ( 0.000000000000000000, -1.000000000000000000, 0.000000000000000000 ) ) ;
#10870=CARTESIAN_POINT ( 'NONE',  ( 96.29968967959054282, 25.52935533987996664, -33.00000000000012790 ) ) ;
#10894=DIRECTION ( 'NONE',  ( -1.000000000000000000, -1.110223024625156540E-15, 0.000000000000000000 ) ) ;
#10930=DIRECTION ( 'NONE',  ( 0.000000000000000000, 1.000000000000000000, -0.000000000000000000 ) ) ;
#10947=SHAPE_DEFINITION_REPRESENTATION ( #4244, #2449 ) ;
#10950=CARTESIAN_POINT ( 'NONE',  ( 64.90552635791956959, 22.43695620243006772, 84.20452624982236500 ) ) ;
#10962=DIRECTION ( 'NONE',  ( 0.000000000000000000, 1.000000000000000000, -0.000000000000000000 ) ) ;
#10982=LINE ( 'NONE', #440, #10765 ) ;
#11005=PRODUCT_DEFINITION_FORMATION_WITH_SPECIFIED_SOURCE ( 'ANY', '', #13583, .NOT_KNOWN. ) ;
#11012=ORIENTED_EDGE ( 'NONE', *, *, #11188, .F. ) ;
#11089=AXIS2_PLACEMENT_3D ( 'NONE', #5447, #5605, #3290 ) ;
#11094=LINE ( 'NONE', #480, #8632 ) ;
#11096=DIRECTION ( 'NONE',  ( 1.000000000000000000, 0.000000000000000000, 0.000000000000000000 ) ) ;
#11136=CARTESIAN_POINT ( 'NONE',  ( 64.90552635791956959, 22.43695620243006772, 84.20452624982236500 ) ) ;
#11174=ORIENTED_EDGE ( 'NONE', *, *, #5087, .T. ) ;
#11188=EDGE_CURVE ( 'NONE', #4627, #1474, #9468, .T. ) ;
#11190=CLOSED_SHELL ( 'NONE', ( #7868, #3008, #654, #8166, #14682, #1387, #9657, #7487, #14856, #3528, #2951, #123, #12507, #15101, #2942, #9854, #5171, #10054 ) ) ;
#11333=LINE ( 'NONE', #5510, #2276 ) ;
#11338=EDGE_CURVE ( 'NONE', #11898, #619, #6161, .T. ) ;
#11430=VERTEX_POINT ( 'NONE', #734 ) ;
#11495=LINE ( 'NONE', #5352, #4360 ) ;
#11522=ORIENTED_EDGE ( 'NONE', *, *, #1739, .F. ) ;
#11523=LINE ( 'NONE', #6607, #1538 ) ;
#11532=LINE ( 'NONE', #14167, #13707 ) ;
#11583=VECTOR ( 'NONE', #11881, 1000.000000000000000 ) ;
#11601=ORIENTED_EDGE ( 'NONE', *, *, #5311, .T. ) ;
#11612=FACE_OUTER_BOUND ( 'NONE', #11, .T. ) ;
#11617=CARTESIAN_POINT ( 'NONE',  ( 80.18290120114222930, 23.25070940071369208, -33.00000000000012790 ) ) ;
#11627=ORIENTED_EDGE ( 'NONE', *, *, #3690, .T. ) ;
#11631=EDGE_CURVE ( 'NONE', #14830, #6001, #3723, .T. ) ;
#11654=( NAMED_UNIT ( * ) PLANE_ANGLE_UNIT ( ) SI_UNIT ( $, .RADIAN. ) );
#11663=UNCERTAINTY_MEASURE_WITH_UNIT (LENGTH_MEASURE( 1.000000000000000082E-05 ), #14044, 'distance_accuracy_value', 'NONE');
#11667=DIRECTION ( 'NONE',  ( 0.000000000000000000, 1.000000000000000000, 0.000000000000000000 ) ) ;
#11672=LINE ( 'NONE', #2363, #12195 ) ;
#11696=CARTESIAN_POINT ( 'NONE',  ( 47.27423575335444639, 23.25070940071368852, -33.00000000000012790 ) ) ;
#11705=ORIENTED_EDGE ( 'NONE', *, *, #13097, .F. ) ;
#11717=DIRECTION ( 'NONE',  ( 0.000000000000000000, 0.000000000000000000, -1.000000000000000000 ) ) ;
#11718=AXIS2_PLACEMENT_3D ( 'NONE', #14143, #3591, #8454 ) ;
#11757=DIRECTION ( 'NONE',  ( -0.000000000000000000, -0.000000000000000000, -1.000000000000000000 ) ) ;
#11784=ORIENTED_EDGE ( 'NONE', *, *, #949, .T. ) ;
#11830=MECHANICAL_DESIGN_GEOMETRIC_PRESENTATION_REPRESENTATION('',(#1004),#14769);
#11834=ORIENTED_EDGE ( 'NONE', *, *, #10349, .T. ) ;
#11843=ORIENTED_EDGE ( 'NONE', *, *, #9277, .T. ) ;
#11863=ORIENTED_EDGE ( 'NONE', *, *, #13097, .T. ) ;
#11881=DIRECTION ( 'NONE',  ( 0.000000000000000000, 1.000000000000000000, -0.000000000000000000 ) ) ;
#11898=VERTEX_POINT ( 'NONE', #7951 ) ;
#11913=DIRECTION ( 'NONE',  ( -0.000000000000000000, -0.000000000000000000, -1.000000000000000000 ) ) ;
#11985=VECTOR ( 'NONE', #11757, 1000.000000000000000 ) ;
#11999=DIRECTION ( 'NONE',  ( 0.000000000000000000, 0.000000000000000000, -1.000000000000000000 ) ) ;
#12055=VECTOR ( 'NONE', #7569, 1000.000000000000000 ) ;
#12057=CARTESIAN_POINT ( 'NONE',  ( 80.18290120114222930, 25.52935533987996664, 33.00000000000012790 ) ) ;
#12093=ORIENTED_EDGE ( 'NONE', *, *, #5326, .T. ) ;
#12097=DIRECTION ( 'NONE',  ( -1.000000000000000000, 0.000000000000000000, 0.000000000000000000 ) ) ;
#12107=EDGE_CURVE ( 'NONE', #6772, #750, #8698, .T. ) ;
#12118=DIRECTION ( 'NONE',  ( 0.000000000000000000, -0.000000000000000000, -1.000000000000000000 ) ) ;
#12120=ORIENTED_EDGE ( 'NONE', *, *, #8626, .T. ) ;
#12164=PRODUCT_CONTEXT ( 'NONE', #2443, 'mechanical' ) ;
#12177=DIRECTION ( 'NONE',  ( 1.000000000000000000, -0.000000000000000000, 0.000000000000000000 ) ) ;
#12192=DIRECTION ( 'NONE',  ( -1.000000000000000000, 0.000000000000000000, 0.000000000000000000 ) ) ;
#12195=VECTOR ( 'NONE', #13904, 1000.000000000000000 ) ;
#12242=CARTESIAN_POINT ( 'NONE',  ( 80.18290120114222930, 23.25070940071369208, 33.00000000000012790 ) ) ;
#12252=FACE_OUTER_BOUND ( 'NONE', #2023, .T. ) ;
#12279=FACE_OUTER_BOUND ( 'NONE', #8596, .T. ) ;
#12281=ORIENTED_EDGE ( 'NONE', *, *, #9241, .T. ) ;
#12316=VERTEX_POINT ( 'NONE', #9471 ) ;
#12322=CARTESIAN_POINT ( 'NONE',  ( 47.27423575335444639, 25.52935533987996664, 84.20452624982236500 ) ) ;
#12343=ORIENTED_EDGE ( 'NONE', *, *, #13654, .T. ) ;
#12413=PLANE ( 'NONE',  #14730 ) ;
#12420=CARTESIAN_POINT ( 'NONE',  ( 82.49066175147797253, 12.46743062497963450, 84.20452624982236500 ) ) ;
#12507=ADVANCED_FACE ( 'NONE', ( #14832 ), #7835, .F. ) ;
#12561=( LENGTH_UNIT ( ) NAMED_UNIT ( * ) SI_UNIT ( .MILLI., .METRE. ) );
#12599=ORIENTED_EDGE ( 'NONE', *, *, #969, .T. ) ;
#12640=DIRECTION ( 'NONE',  ( 1.000000000000000000, -0.000000000000000000, 0.000000000000000000 ) ) ;
#12642=VERTEX_POINT ( 'NONE', #8654 ) ;
#12718=( NAMED_UNIT ( * ) SI_UNIT ( $, .STERADIAN. ) SOLID_ANGLE_UNIT ( ) );
#12794=VECTOR ( 'NONE', #11913, 1000.000000000000000 ) ;
#12832=VECTOR ( 'NONE', #15119, 1000.000000000000000 ) ;
#12902=CARTESIAN_POINT ( 'NONE',  ( 47.27423575335444639, 25.52935533987996664, 84.20452624982236500 ) ) ;
#13007=ORIENTED_EDGE ( 'NONE', *, *, #5326, .F. ) ;
#13083=ORIENTED_EDGE ( 'NONE', *, *, #13984, .T. ) ;
#13097=EDGE_CURVE ( 'NONE', #12316, #4627, #11523, .T. ) ;
#13108=AXIS2_PLACEMENT_3D ( 'NONE', #14201, #10582, #10505 ) ;
#13138=FACE_OUTER_BOUND ( 'NONE', #15064, .T. ) ;
#13225=ORIENTED_EDGE ( 'NONE', *, *, #5053, .F. ) ;
#13259=CARTESIAN_POINT ( 'NONE',  ( 96.29968967959054282, 23.25070940071369208, 33.00000000000012790 ) ) ;
#13266=LINE ( 'NONE', #5034, #9594 ) ;
#13285=ORIENTED_EDGE ( 'NONE', *, *, #4021, .F. ) ;
#13293=ORIENTED_EDGE ( 'NONE', *, *, #13984, .F. ) ;
#13361=VECTOR ( 'NONE', #10930, 1000.000000000000000 ) ;
#13437=FACE_OUTER_BOUND ( 'NONE', #6137, .T. ) ;
#13451=CARTESIAN_POINT ( 'NONE',  ( 96.29968967959054282, 23.25070940071369208, -33.00000000000012790 ) ) ;
#13467=AXIS2_PLACEMENT_3D ( 'NONE', #14608, #4059, #8757 ) ;
#13493=DIRECTION ( 'NONE',  ( 0.000000000000000000, 1.000000000000000000, -0.000000000000000000 ) ) ;
#13560=EDGE_LOOP ( 'NONE', ( #14562, #11843, #4818, #8297 ) ) ;
#13565=FACE_OUTER_BOUND ( 'NONE', #479, .T. ) ;
#13583=PRODUCT ( 'Small Aluminum Top-Plate Insert', 'Small Aluminum Top-Plate Insert', '', ( #12164 ) ) ;
#13605=CARTESIAN_POINT ( 'NONE',  ( 67.21328690825531282, 22.43695620243006772, 33.00000000000012790 ) ) ;
#13629=ORIENTED_EDGE ( 'NONE', *, *, #9277, .F. ) ;
#13654=EDGE_CURVE ( 'NONE', #1474, #788, #9289, .T. ) ;
#13662=CARTESIAN_POINT ( 'NONE',  ( 58.92629142760364402, 23.25070940071368852, 33.00000000000012790 ) ) ;
#13707=VECTOR ( 'NONE', #15164, 1000.000000000000000 ) ;
#13770=LINE ( 'NONE', #4222, #6950 ) ;
#13826=DIRECTION ( 'NONE',  ( -1.000000000000000000, 0.000000000000000000, 0.000000000000000000 ) ) ;
#13880=ORIENTED_EDGE ( 'NONE', *, *, #14128, .T. ) ;
#13904=DIRECTION ( 'NONE',  ( -1.000000000000000000, 0.000000000000000000, 0.000000000000000000 ) ) ;
#13908=CARTESIAN_POINT ( 'NONE',  ( 82.49066175147797253, 23.25070940071369208, 84.20452624982236500 ) ) ;
#13975=VECTOR ( 'NONE', #1347, 1000.000000000000000 ) ;
#13980=UNCERTAINTY_MEASURE_WITH_UNIT (LENGTH_MEASURE( 1.000000000000000082E-05 ), #12561, 'distance_accuracy_value', 'NONE');
#13984=EDGE_CURVE ( 'NONE', #5864, #9890, #9199, .T. ) ;
#13995=VECTOR ( 'NONE', #5646, 1000.000000000000000 ) ;
#14002=EDGE_CURVE ( 'NONE', #14996, #11430, #1339, .T. ) ;
#14030=DIRECTION ( 'NONE',  ( 0.000000000000000000, 1.000000000000000000, 0.000000000000000000 ) ) ;
#14044=( LENGTH_UNIT ( ) NAMED_UNIT ( * ) SI_UNIT ( .MILLI., .METRE. ) );
#14073=EDGE_CURVE ( 'NONE', #12316, #6772, #1101, .T. ) ;
#14128=EDGE_CURVE ( 'NONE', #619, #5990, #11094, .T. ) ;
#14143=CARTESIAN_POINT ( 'NONE',  ( 96.29968967959054282, 23.25070940071369208, 84.20452624982236500 ) ) ;
#14160=DIRECTION ( 'NONE',  ( 0.000000000000000000, 0.000000000000000000, 1.000000000000000000 ) ) ;
#14167=CARTESIAN_POINT ( 'NONE',  ( 80.18290120114222930, 23.25070940071369208, -33.00000000000012790 ) ) ;
#14186=VECTOR ( 'NONE', #1158, 1000.000000000000000 ) ;
#14201=CARTESIAN_POINT ( 'NONE',  ( 88.00000000000001421, 10.75070940071369208, 84.20452624982236500 ) ) ;
#14217=ORIENTED_EDGE ( 'NONE', *, *, #1739, .T. ) ;
#14227=ORIENTED_EDGE ( 'NONE', *, *, #1969, .F. ) ;
#14228=VERTEX_POINT ( 'NONE', #8860 ) ;
#14233=CARTESIAN_POINT ( 'NONE',  ( 67.21328690825531282, 22.43695620243006772, 84.20452624982236500 ) ) ;
#14270=DIRECTION ( 'NONE',  ( -0.000000000000000000, -0.000000000000000000, -1.000000000000000000 ) ) ;
#14284=EDGE_LOOP ( 'NONE', ( #2981, #12599, #1516, #13629 ) ) ;
#14299=VECTOR ( 'NONE', #11717, 1000.000000000000000 ) ;
#14354=EDGE_LOOP ( 'NONE', ( #1215, #5913, #1541, #1899 ) ) ;
#14379=CARTESIAN_POINT ( 'NONE',  ( 64.90552635791956959, 22.43695620243006772, 33.00000000000014211 ) ) ;
#14395=DIRECTION ( 'NONE',  ( 1.000000000000000000, 0.000000000000000000, 0.000000000000000000 ) ) ;
#14429=PLANE ( 'NONE',  #275 ) ;
#14505=ORIENTED_EDGE ( 'NONE', *, *, #7226, .T. ) ;
#14562=ORIENTED_EDGE ( 'NONE', *, *, #5087, .F. ) ;
#14608=CARTESIAN_POINT ( 'NONE',  ( 67.21328690825531282, 22.43695620243006772, 84.20452624982236500 ) ) ;
#14632=VECTOR ( 'NONE', #7403, 1000.000000000000000 ) ;
#14634=ORIENTED_EDGE ( 'NONE', *, *, #11338, .T. ) ;
#14648=DIRECTION ( 'NONE',  ( 0.000000000000000000, 0.000000000000000000, -1.000000000000000000 ) ) ;
#14651=ORIENTED_EDGE ( 'NONE', *, *, #12107, .F. ) ;
#14682=ADVANCED_FACE ( 'NONE', ( #10677 ), #212, .F. ) ;
#14722=CARTESIAN_POINT ( 'NONE',  ( 82.49066175147797253, 23.25070940071369208, 84.20452624982236500 ) ) ;
#14730=AXIS2_PLACEMENT_3D ( 'NONE', #14722, #13493, #3038 ) ;
#14753=DIRECTION ( 'NONE',  ( 0.000000000000000000, -1.000000000000000000, 0.000000000000000000 ) ) ;
#14754=EDGE_CURVE ( 'NONE', #6995, #3172, #6219, .T. ) ;
#14769=( GEOMETRIC_REPRESENTATION_CONTEXT ( 3 ) GLOBAL_UNCERTAINTY_ASSIGNED_CONTEXT ( ( #11663 ) ) GLOBAL_UNIT_ASSIGNED_CONTEXT ( ( #14044, #11654, #10585 ) ) REPRESENTATION_CONTEXT ( 'NONE', 'WORKASPACE' ) );
#14802=VECTOR ( 'NONE', #12097, 1000.000000000000000 ) ;
#14815=DIRECTION ( 'NONE',  ( 0.000000000000000000, -1.000000000000000000, 0.000000000000000000 ) ) ;
#14826=PLANE ( 'NONE',  #630 ) ;
#14830=VERTEX_POINT ( 'NONE', #5127 ) ;
#14832=FACE_OUTER_BOUND ( 'NONE', #14843, .T. ) ;
#14839=CARTESIAN_POINT ( 'NONE',  ( 47.27423575335444639, 25.52935533987996664, -33.00000000000012790 ) ) ;
#14843=EDGE_LOOP ( 'NONE', ( #1930, #7471, #4771, #13285 ) ) ;
#14852=EDGE_CURVE ( 'NONE', #788, #4378, #8657, .T. ) ;
#14856=ADVANCED_FACE ( 'NONE', ( #497 ), #5747, .F. ) ;
#14857=DIRECTION ( 'NONE',  ( 1.000000000000000000, 1.156482317317871725E-16, -0.000000000000000000 ) ) ;
#14868=CARTESIAN_POINT ( 'NONE',  ( 47.27423575335444639, 23.25070940071368852, -33.00000000000012790 ) ) ;
#14873=ORIENTED_EDGE ( 'NONE', *, *, #8949, .T. ) ;
#14888=EDGE_CURVE ( 'NONE', #2618, #5069, #11333, .T. ) ;
#14912=AXIS2_PLACEMENT_3D ( 'NONE', #4039, #9913, #7745 ) ;
#14964=EDGE_CURVE ( 'NONE', #3249, #1474, #10196, .T. ) ;
#14996=VERTEX_POINT ( 'NONE', #9202 ) ;
#15010=AXIS2_PLACEMENT_3D ( 'NONE', #9744, #2722, #12118 ) ;
#15018=LINE ( 'NONE', #3087, #5671 ) ;
#15064=EDGE_LOOP ( 'NONE', ( #8195, #4024, #9160, #13293 ) ) ;
#15101=ADVANCED_FACE ( 'NONE', ( #7036 ), #6043, .F. ) ;
#15119=DIRECTION ( 'NONE',  ( -0.000000000000000000, -0.000000000000000000, -1.000000000000000000 ) ) ;
#15138=LINE ( 'NONE', #5767, #171 ) ;
#15164=DIRECTION ( 'NONE',  ( 0.000000000000000000, 1.000000000000000000, 0.000000000000000000 ) ) ;
#15189=LINE ( 'NONE', #6787, #13995 ) ;
#15203=CARTESIAN_POINT ( 'NONE',  ( 96.29968967959054282, 25.52935533987996664, 84.20452624982236500 ) ) ;
#15273=COLOUR_RGB('Off White',0.89,0.88,0.83);
#15274=FILL_AREA_STYLE_COLOUR('',#15273);
#15275=FILL_AREA_STYLE('',(#15274));
#15276=SURFACE_STYLE_FILL_AREA(#15275);
#15277=SURFACE_SIDE_STYLE('',(#15276));
#15278=SURFACE_STYLE_USAGE(.BOTH.,#15277);
#15279=PRESENTATION_STYLE_ASSIGNMENT((#15278));
ENDSEC;
END-ISO-10303-21;
